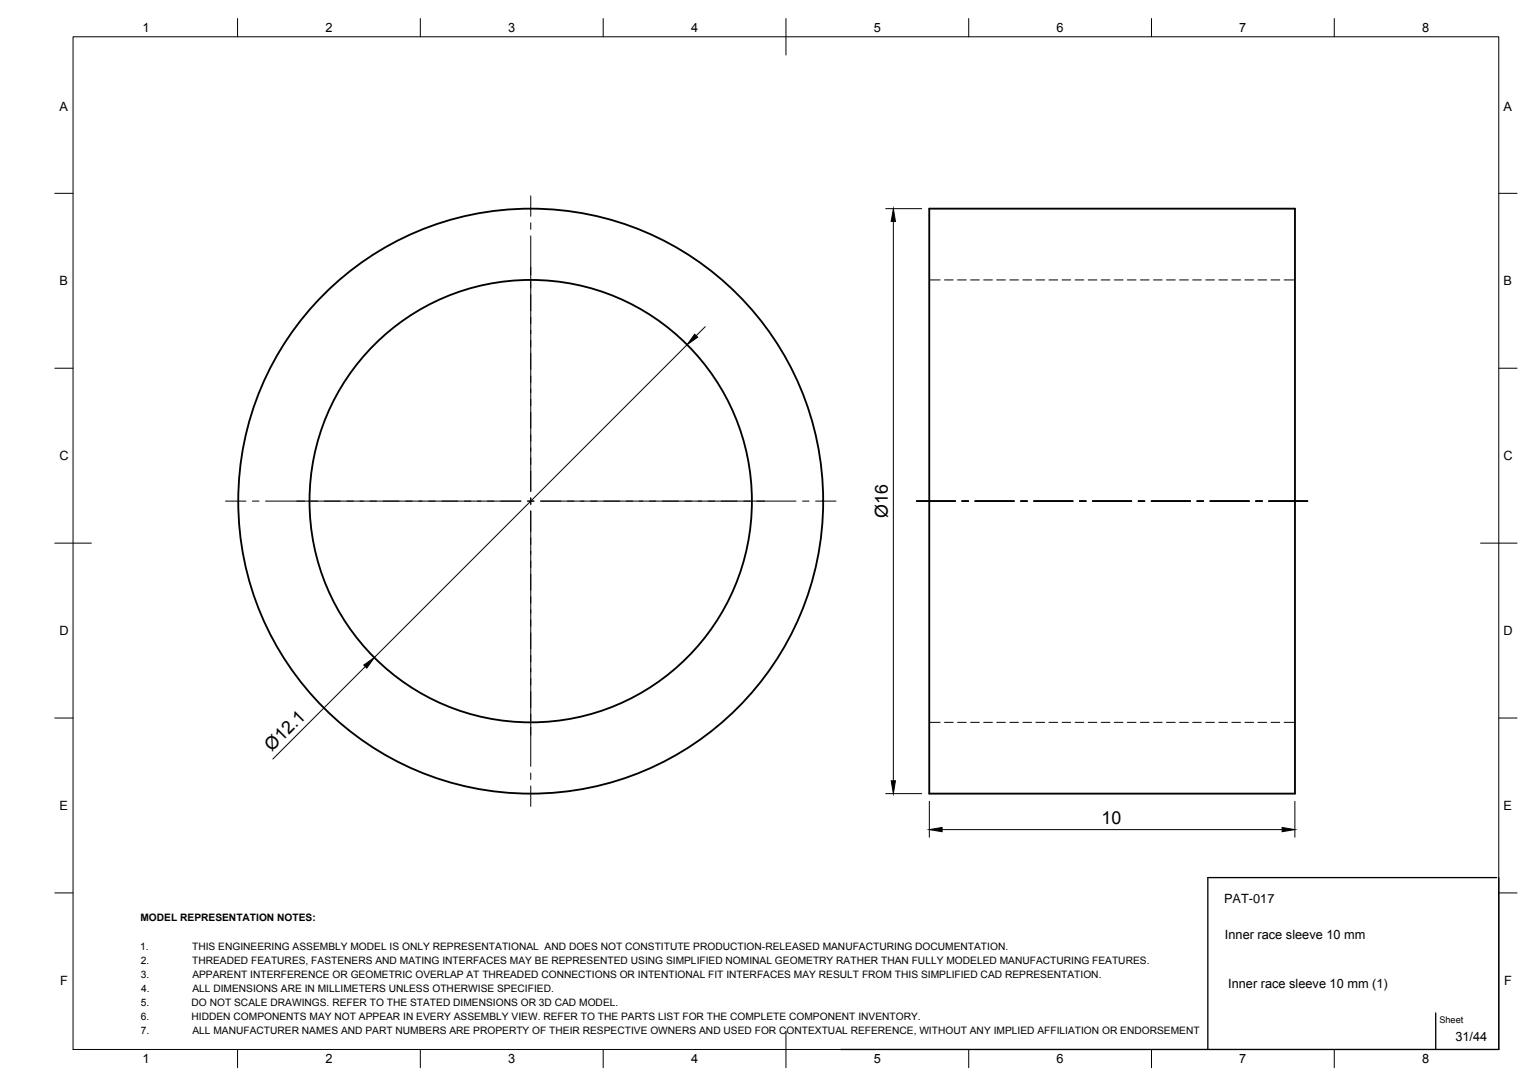
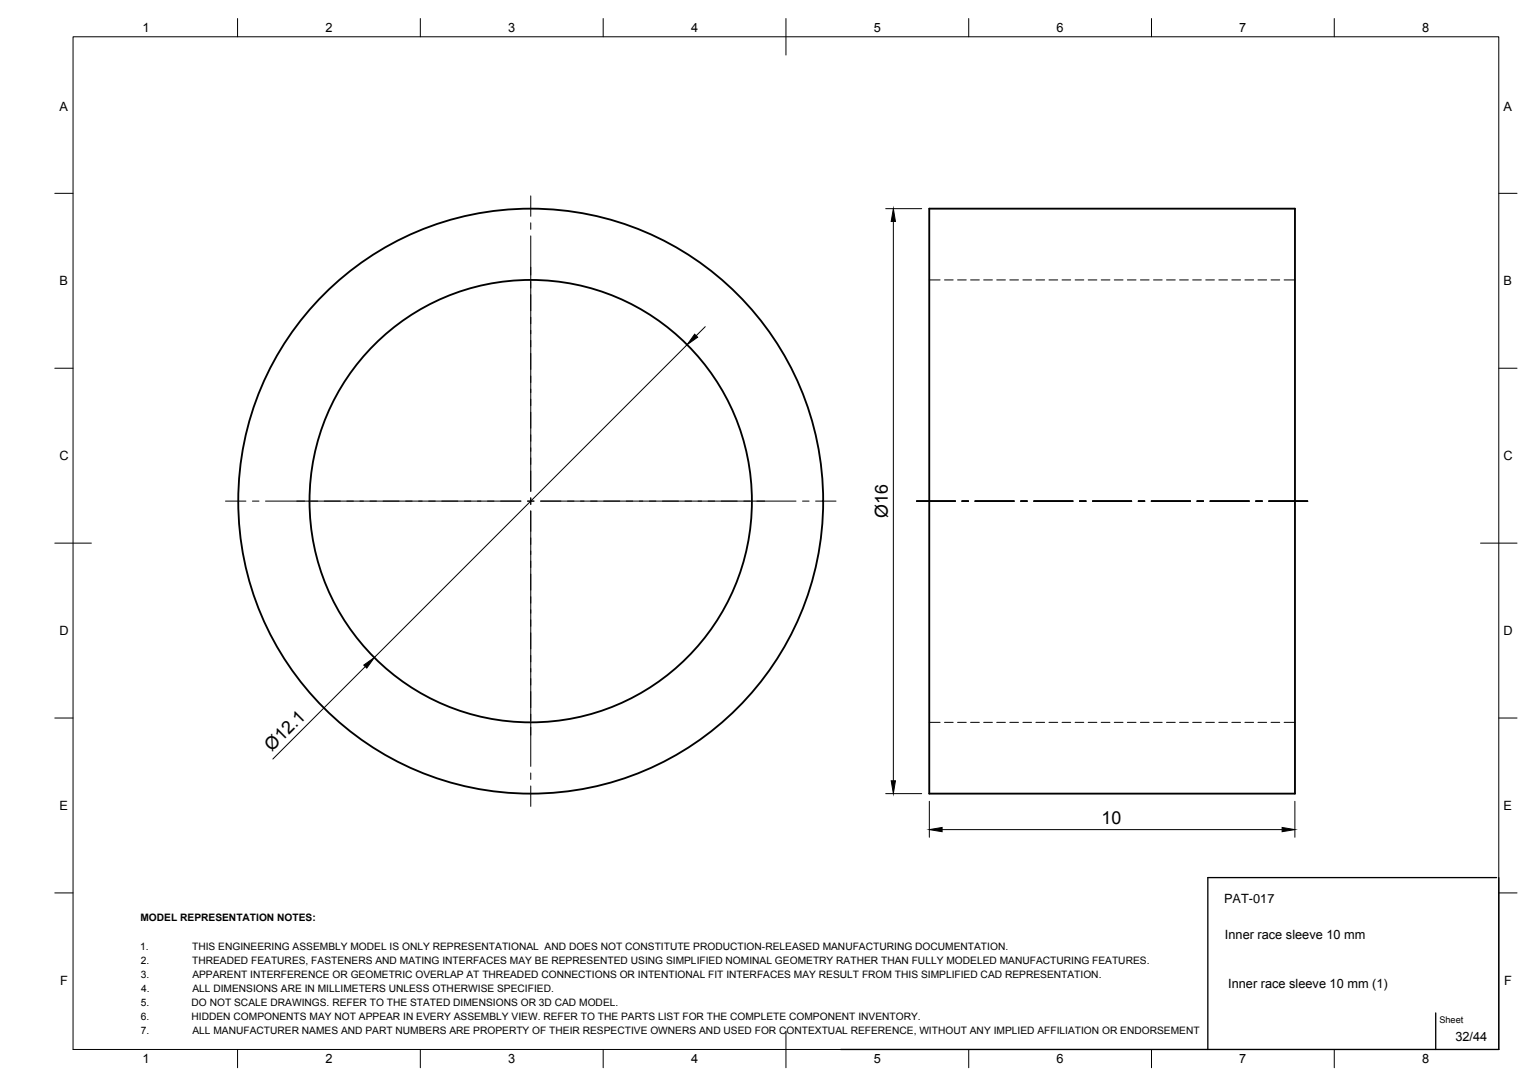
ISO-10303-21;
HEADER;
/* Generated by software containing ST-Developer
 * from STEP Tools, Inc. (www.steptools.com) 
 */

FILE_DESCRIPTION(
/* description */ ('Cam-and-follower valve demonstrator'),
/* implementation_level */ '2;1');

FILE_NAME(
/* name */ 'Inner race sleeve 10 mm.step',
/* time_stamp */ '2026-10-28T03:25:17-07:00',
/* author */ (''),
/* organization */ (''),
/* preprocessor_version */ 'ST-DEVELOPER v20.2',
/* originating_system */ 'Autodesk Translation Framework v15.17.0.0',
/* authorisation */ '');

FILE_SCHEMA (('AUTOMOTIVE_DESIGN { 1 0 10303 214 3 1 1 }'));
ENDSEC;

DATA;
#10=MECHANICAL_DESIGN_GEOMETRIC_PRESENTATION_REPRESENTATION('',(#441),#12896);
#362=SHAPE_REPRESENTATION_RELATIONSHIP('SRR','None',#13081,#398);
#398=ADVANCED_BREP_SHAPE_REPRESENTATION('',(#482),#12881);
#441=STYLED_ITEM('',(#13330),#482);
#482=MANIFOLD_SOLID_BREP('Body1',#6210);
#630=FACE_BOUND('',#1871,.T.);
#631=FACE_BOUND('',#1873,.T.);
#907=CIRCLE('',#7175,0.605);
#908=CIRCLE('',#7176,0.605);
#909=CIRCLE('',#7178,0.8);
#910=CIRCLE('',#7179,0.8);
#1065=CYLINDRICAL_SURFACE('',#7174,0.605);
#1066=CYLINDRICAL_SURFACE('',#7177,0.8);
#1365=FACE_OUTER_BOUND('',#1868,.T.);
#1366=FACE_OUTER_BOUND('',#1869,.T.);
#1367=FACE_OUTER_BOUND('',#1870,.T.);
#1368=FACE_OUTER_BOUND('',#1872,.T.);
#1868=EDGE_LOOP('',(#5239,#5240,#5241,#5242));
#1869=EDGE_LOOP('',(#5243,#5244,#5245,#5246));
#1870=EDGE_LOOP('',(#5247));
#1871=EDGE_LOOP('',(#5248));
#1872=EDGE_LOOP('',(#5249));
#1873=EDGE_LOOP('',(#5250));
#2304=LINE('',#12344,#2726);
#2305=LINE('',#12350,#2727);
#2726=VECTOR('',#8831,0.605);
#2727=VECTOR('',#8838,0.8);
#3226=VERTEX_POINT('',#12341);
#3227=VERTEX_POINT('',#12343);
#3228=VERTEX_POINT('',#12347);
#3229=VERTEX_POINT('',#12349);
#3916=EDGE_CURVE('',#3226,#3226,#907,.T.);
#3917=EDGE_CURVE('',#3226,#3227,#2304,.T.);
#3918=EDGE_CURVE('',#3227,#3227,#908,.T.);
#3919=EDGE_CURVE('',#3228,#3228,#909,.T.);
#3920=EDGE_CURVE('',#3228,#3229,#2305,.T.);
#3921=EDGE_CURVE('',#3229,#3229,#910,.T.);
#5239=ORIENTED_EDGE('',*,*,#3916,.F.);
#5240=ORIENTED_EDGE('',*,*,#3917,.T.);
#5241=ORIENTED_EDGE('',*,*,#3918,.T.);
#5242=ORIENTED_EDGE('',*,*,#3917,.F.);
#5243=ORIENTED_EDGE('',*,*,#3919,.F.);
#5244=ORIENTED_EDGE('',*,*,#3920,.T.);
#5245=ORIENTED_EDGE('',*,*,#3921,.T.);
#5246=ORIENTED_EDGE('',*,*,#3920,.F.);
#5247=ORIENTED_EDGE('',*,*,#3919,.T.);
#5248=ORIENTED_EDGE('',*,*,#3916,.T.);
#5249=ORIENTED_EDGE('',*,*,#3921,.F.);
#5250=ORIENTED_EDGE('',*,*,#3918,.F.);
#5747=PLANE('',#7180);
#5748=PLANE('',#7181);
#6081=ADVANCED_FACE('',(#1365),#1065,.F.);
#6082=ADVANCED_FACE('',(#1366),#1066,.T.);
#6083=ADVANCED_FACE('',(#1367,#630),#5747,.T.);
#6084=ADVANCED_FACE('',(#1368,#631),#5748,.F.);
#6210=CLOSED_SHELL('',(#6081,#6082,#6083,#6084));
#7173=AXIS2_PLACEMENT_3D('',#12339,#8825,#8826);
#7174=AXIS2_PLACEMENT_3D('',#12340,#8827,#8828);
#7175=AXIS2_PLACEMENT_3D('',#12342,#8829,#8830);
#7176=AXIS2_PLACEMENT_3D('',#12345,#8832,#8833);
#7177=AXIS2_PLACEMENT_3D('',#12346,#8834,#8835);
#7178=AXIS2_PLACEMENT_3D('',#12348,#8836,#8837);
#7179=AXIS2_PLACEMENT_3D('',#12351,#8839,#8840);
#7180=AXIS2_PLACEMENT_3D('',#12352,#8841,#8842);
#7181=AXIS2_PLACEMENT_3D('',#12353,#8843,#8844);
#8825=DIRECTION('axis',(0.,0.,1.));
#8826=DIRECTION('refdir',(1.,0.,0.));
#8827=DIRECTION('center_axis',(0.,1.,0.));
#8828=DIRECTION('ref_axis',(1.,0.,0.));
#8829=DIRECTION('center_axis',(0.,-1.,0.));
#8830=DIRECTION('ref_axis',(1.,0.,0.));
#8831=DIRECTION('',(0.,-1.,0.));
#8832=DIRECTION('center_axis',(0.,-1.,0.));
#8833=DIRECTION('ref_axis',(1.,0.,0.));
#8834=DIRECTION('center_axis',(0.,1.,0.));
#8835=DIRECTION('ref_axis',(1.,0.,0.));
#8836=DIRECTION('center_axis',(0.,1.,0.));
#8837=DIRECTION('ref_axis',(1.,0.,0.));
#8838=DIRECTION('',(0.,-1.,0.));
#8839=DIRECTION('center_axis',(0.,1.,0.));
#8840=DIRECTION('ref_axis',(1.,0.,0.));
#8841=DIRECTION('center_axis',(0.,1.,0.));
#8842=DIRECTION('ref_axis',(1.,0.,0.));
#8843=DIRECTION('center_axis',(0.,1.,0.));
#8844=DIRECTION('ref_axis',(1.,0.,0.));
#12339=CARTESIAN_POINT('',(0.,0.,0.));
#12340=CARTESIAN_POINT('Origin',(0.,-2.,4.));
#12341=CARTESIAN_POINT('',(-0.605,-1.,4.));
#12342=CARTESIAN_POINT('Origin',(0.,-1.,4.));
#12343=CARTESIAN_POINT('',(-0.605,-2.,4.));
#12344=CARTESIAN_POINT('',(-0.605,-2.,4.));
#12345=CARTESIAN_POINT('Origin',(0.,-2.,4.));
#12346=CARTESIAN_POINT('Origin',(0.,-2.,4.));
#12347=CARTESIAN_POINT('',(-0.8,-1.,4.));
#12348=CARTESIAN_POINT('Origin',(0.,-1.,4.));
#12349=CARTESIAN_POINT('',(-0.8,-2.,4.));
#12350=CARTESIAN_POINT('',(-0.8,-2.,4.));
#12351=CARTESIAN_POINT('Origin',(0.,-2.,4.));
#12352=CARTESIAN_POINT('Origin',(0.,-1.,4.));
#12353=CARTESIAN_POINT('Origin',(0.,-2.,4.));
#12838=UNCERTAINTY_MEASURE_WITH_UNIT(LENGTH_MEASURE(0.001),#12897,
'DISTANCE_ACCURACY_VALUE',
'Maximum model space distance between geometric entities at asserted c
onnectivities');
#12853=UNCERTAINTY_MEASURE_WITH_UNIT(LENGTH_MEASURE(0.001),#12897,
'DISTANCE_ACCURACY_VALUE',
'Maximum model space distance between geometric entities at asserted c
onnectivities');
#12881=(
GEOMETRIC_REPRESENTATION_CONTEXT(3)
GLOBAL_UNCERTAINTY_ASSIGNED_CONTEXT((#12838))
GLOBAL_UNIT_ASSIGNED_CONTEXT((#12897,#12899,#12900))
REPRESENTATION_CONTEXT('','3D')
);
#12896=(
GEOMETRIC_REPRESENTATION_CONTEXT(3)
GLOBAL_UNCERTAINTY_ASSIGNED_CONTEXT((#12853))
GLOBAL_UNIT_ASSIGNED_CONTEXT((#12897,#12899,#12900))
REPRESENTATION_CONTEXT('','3D')
);
#12897=(
LENGTH_UNIT()
NAMED_UNIT(*)
SI_UNIT(.CENTI.,.METRE.)
);
#12899=(
NAMED_UNIT(*)
PLANE_ANGLE_UNIT()
SI_UNIT($,.RADIAN.)
);
#12900=(
NAMED_UNIT(*)
SI_UNIT($,.STERADIAN.)
SOLID_ANGLE_UNIT()
);
#12928=SHAPE_DEFINITION_REPRESENTATION(#12977,#13081);
#12977=PRODUCT_DEFINITION_SHAPE('',$,#13124);
#13081=SHAPE_REPRESENTATION('',(#7173),#12881);
#13096=PRODUCT_DEFINITION_CONTEXT('part definition',#13224,'design');
#13124=PRODUCT_DEFINITION('Inner race sleeve 10 mm',
'Inner race sleeve 10 mm',#13166,#13096);
#13166=PRODUCT_DEFINITION_FORMATION('',$,#13253);
#13224=APPLICATION_CONTEXT(
'Core Data for Automotive Mechanical Design Process');
#13225=PRODUCT_CONTEXT('part definition',#13224,'mechanical');
#13253=PRODUCT('Inner race sleeve 10 mm','Inner race sleeve 10 mm',
'Inner race sleeve 10 mm',(#13225));
#13324=COLOUR_RGB('Grey',0.48,0.52,0.57);
#13325=FILL_AREA_STYLE_COLOUR('',#13324);
#13326=FILL_AREA_STYLE('',(#13325));
#13327=SURFACE_STYLE_FILL_AREA(#13326);
#13328=SURFACE_SIDE_STYLE('',(#13327));
#13329=SURFACE_STYLE_USAGE(.BOTH.,#13328);
#13330=PRESENTATION_STYLE_ASSIGNMENT((#13329));
ENDSEC;
END-ISO-10303-21;
